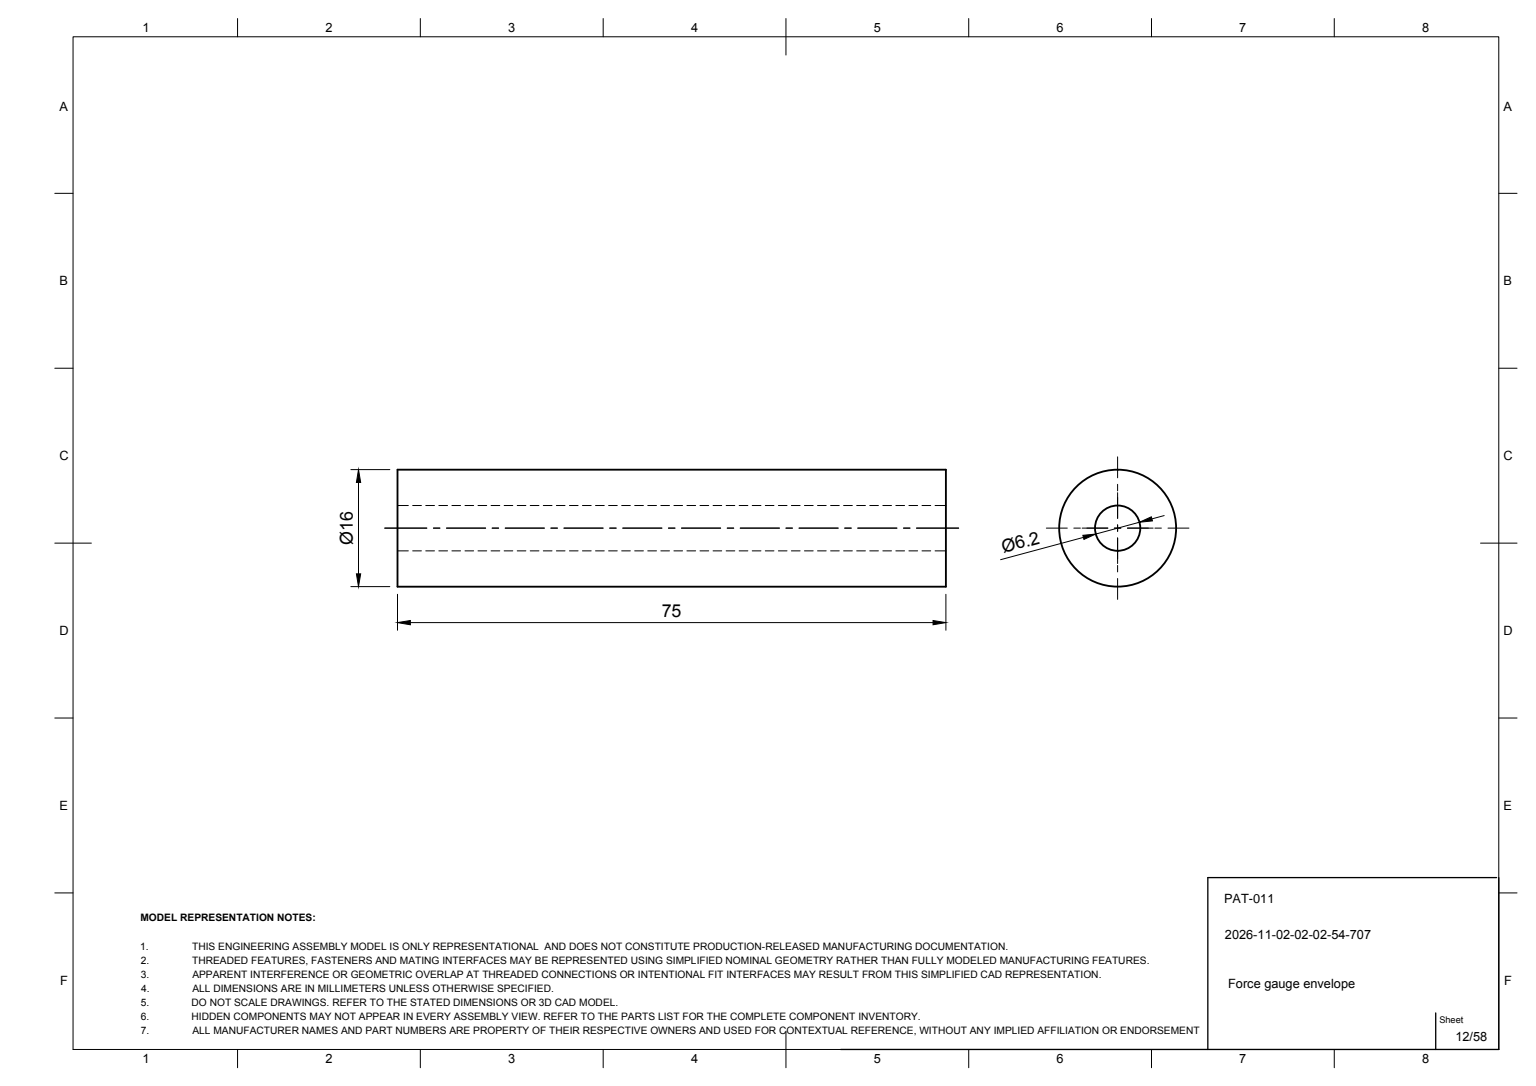
ISO-10303-21;
HEADER;
/* Generated by software containing ST-Developer
 * from STEP Tools, Inc. (www.steptools.com) 
 */

FILE_DESCRIPTION(
/* description */ ('Belt tension measurement rig'),
/* implementation_level */ '2;1');

FILE_NAME(
/* name */ 'Force gauge envelope.step',
/* time_stamp */ '2026-10-28T03:24:44-07:00',
/* author */ (''),
/* organization */ (''),
/* preprocessor_version */ 'ST-DEVELOPER v20.2',
/* originating_system */ 'Autodesk Translation Framework v15.17.0.0',
/* authorisation */ '');

FILE_SCHEMA (('AUTOMOTIVE_DESIGN { 1 0 10303 214 3 1 1 }'));
ENDSEC;

DATA;
#10=MECHANICAL_DESIGN_GEOMETRIC_PRESENTATION_REPRESENTATION('',(#703),#23587);
#593=SHAPE_REPRESENTATION_RELATIONSHIP('SRR','None',#23838,#648);
#648=ADVANCED_BREP_SHAPE_REPRESENTATION('',(#773),#23536);
#703=STYLED_ITEM('',(#24225),#773);
#773=MANIFOLD_SOLID_BREP('Body1',#12208);
#889=FACE_BOUND('',#2248,.T.);
#890=FACE_BOUND('',#2250,.T.);
#1107=PLANE('',#13143);
#1108=PLANE('',#13144);
#1481=FACE_OUTER_BOUND('',#2245,.T.);
#1482=FACE_OUTER_BOUND('',#2246,.T.);
#1483=FACE_OUTER_BOUND('',#2247,.T.);
#1484=FACE_OUTER_BOUND('',#2249,.T.);
#2245=EDGE_LOOP('',(#8460,#8461,#8462,#8463));
#2246=EDGE_LOOP('',(#8464,#8465,#8466,#8467));
#2247=EDGE_LOOP('',(#8468));
#2248=EDGE_LOOP('',(#8469));
#2249=EDGE_LOOP('',(#8470));
#2250=EDGE_LOOP('',(#8471));
#3111=LINE('',#19132,#3862);
#3112=LINE('',#19138,#3863);
#3862=VECTOR('',#15186,0.31);
#3863=VECTOR('',#15193,0.8);
#4588=CIRCLE('',#13138,0.31);
#4589=CIRCLE('',#13139,0.31);
#4590=CIRCLE('',#13141,0.8);
#4591=CIRCLE('',#13142,0.8);
#5412=VERTEX_POINT('',#19129);
#5413=VERTEX_POINT('',#19131);
#5414=VERTEX_POINT('',#19135);
#5415=VERTEX_POINT('',#19137);
#6589=EDGE_CURVE('',#5412,#5412,#4588,.T.);
#6590=EDGE_CURVE('',#5412,#5413,#3111,.T.);
#6591=EDGE_CURVE('',#5413,#5413,#4589,.T.);
#6592=EDGE_CURVE('',#5414,#5414,#4590,.T.);
#6593=EDGE_CURVE('',#5414,#5415,#3112,.T.);
#6594=EDGE_CURVE('',#5415,#5415,#4591,.T.);
#8460=ORIENTED_EDGE('',*,*,#6589,.F.);
#8461=ORIENTED_EDGE('',*,*,#6590,.T.);
#8462=ORIENTED_EDGE('',*,*,#6591,.T.);
#8463=ORIENTED_EDGE('',*,*,#6590,.F.);
#8464=ORIENTED_EDGE('',*,*,#6592,.F.);
#8465=ORIENTED_EDGE('',*,*,#6593,.T.);
#8466=ORIENTED_EDGE('',*,*,#6594,.T.);
#8467=ORIENTED_EDGE('',*,*,#6593,.F.);
#8468=ORIENTED_EDGE('',*,*,#6592,.T.);
#8469=ORIENTED_EDGE('',*,*,#6589,.T.);
#8470=ORIENTED_EDGE('',*,*,#6594,.F.);
#8471=ORIENTED_EDGE('',*,*,#6591,.F.);
#11217=CYLINDRICAL_SURFACE('',#13137,0.31);
#11218=CYLINDRICAL_SURFACE('',#13140,0.8);
#11622=ADVANCED_FACE('',(#1481),#11217,.F.);
#11623=ADVANCED_FACE('',(#1482),#11218,.T.);
#11624=ADVANCED_FACE('',(#1483,#889),#1107,.T.);
#11625=ADVANCED_FACE('',(#1484,#890),#1108,.F.);
#12208=CLOSED_SHELL('',(#11622,#11623,#11624,#11625));
#13136=AXIS2_PLACEMENT_3D('',#19127,#15180,#15181);
#13137=AXIS2_PLACEMENT_3D('',#19128,#15182,#15183);
#13138=AXIS2_PLACEMENT_3D('',#19130,#15184,#15185);
#13139=AXIS2_PLACEMENT_3D('',#19133,#15187,#15188);
#13140=AXIS2_PLACEMENT_3D('',#19134,#15189,#15190);
#13141=AXIS2_PLACEMENT_3D('',#19136,#15191,#15192);
#13142=AXIS2_PLACEMENT_3D('',#19139,#15194,#15195);
#13143=AXIS2_PLACEMENT_3D('',#19140,#15196,#15197);
#13144=AXIS2_PLACEMENT_3D('',#19141,#15198,#15199);
#15180=DIRECTION('axis',(0.,0.,1.));
#15181=DIRECTION('refdir',(1.,0.,0.));
#15182=DIRECTION('center_axis',(1.,0.,0.));
#15183=DIRECTION('ref_axis',(0.,0.,-1.));
#15184=DIRECTION('center_axis',(-1.,0.,0.));
#15185=DIRECTION('ref_axis',(0.,0.,-1.));
#15186=DIRECTION('',(-1.,0.,0.));
#15187=DIRECTION('center_axis',(-1.,0.,0.));
#15188=DIRECTION('ref_axis',(0.,0.,-1.));
#15189=DIRECTION('center_axis',(1.,0.,0.));
#15190=DIRECTION('ref_axis',(0.,0.,-1.));
#15191=DIRECTION('center_axis',(1.,0.,0.));
#15192=DIRECTION('ref_axis',(0.,0.,-1.));
#15193=DIRECTION('',(-1.,0.,0.));
#15194=DIRECTION('center_axis',(1.,0.,0.));
#15195=DIRECTION('ref_axis',(0.,0.,-1.));
#15196=DIRECTION('center_axis',(1.,0.,0.));
#15197=DIRECTION('ref_axis',(0.,0.,-1.));
#15198=DIRECTION('center_axis',(1.,0.,0.));
#15199=DIRECTION('ref_axis',(0.,0.,-1.));
#19127=CARTESIAN_POINT('',(0.,0.,0.));
#19128=CARTESIAN_POINT('Origin',(2.,7.5,4.5));
#19129=CARTESIAN_POINT('',(9.5,7.5,4.81));
#19130=CARTESIAN_POINT('Origin',(9.5,7.5,4.5));
#19131=CARTESIAN_POINT('',(2.,7.5,4.81));
#19132=CARTESIAN_POINT('',(2.,7.5,4.81));
#19133=CARTESIAN_POINT('Origin',(2.,7.5,4.5));
#19134=CARTESIAN_POINT('Origin',(2.,7.5,4.5));
#19135=CARTESIAN_POINT('',(9.5,7.5,5.3));
#19136=CARTESIAN_POINT('Origin',(9.5,7.5,4.5));
#19137=CARTESIAN_POINT('',(2.,7.5,5.3));
#19138=CARTESIAN_POINT('',(2.,7.5,5.3));
#19139=CARTESIAN_POINT('Origin',(2.,7.5,4.5));
#19140=CARTESIAN_POINT('Origin',(9.5,7.5,4.5));
#19141=CARTESIAN_POINT('Origin',(2.,7.5,4.5));
#23471=UNCERTAINTY_MEASURE_WITH_UNIT(LENGTH_MEASURE(0.001),#23588,
'DISTANCE_ACCURACY_VALUE',
'Maximum model space distance between geometric entities at asserted c
onnectivities');
#23522=UNCERTAINTY_MEASURE_WITH_UNIT(LENGTH_MEASURE(0.001),#23588,
'DISTANCE_ACCURACY_VALUE',
'Maximum model space distance between geometric entities at asserted c
onnectivities');
#23536=(
GEOMETRIC_REPRESENTATION_CONTEXT(3)
GLOBAL_UNCERTAINTY_ASSIGNED_CONTEXT((#23471))
GLOBAL_UNIT_ASSIGNED_CONTEXT((#23588,#23590,#23591))
REPRESENTATION_CONTEXT('','3D')
);
#23587=(
GEOMETRIC_REPRESENTATION_CONTEXT(3)
GLOBAL_UNCERTAINTY_ASSIGNED_CONTEXT((#23522))
GLOBAL_UNIT_ASSIGNED_CONTEXT((#23588,#23590,#23591))
REPRESENTATION_CONTEXT('','3D')
);
#23588=(
LENGTH_UNIT()
NAMED_UNIT(*)
SI_UNIT(.CENTI.,.METRE.)
);
#23590=(
NAMED_UNIT(*)
PLANE_ANGLE_UNIT()
SI_UNIT($,.RADIAN.)
);
#23591=(
NAMED_UNIT(*)
SI_UNIT($,.STERADIAN.)
SOLID_ANGLE_UNIT()
);
#23605=SHAPE_DEFINITION_REPRESENTATION(#23669,#23838);
#23669=PRODUCT_DEFINITION_SHAPE('',$,#23903);
#23838=SHAPE_REPRESENTATION('',(#13136),#23536);
#23889=PRODUCT_DEFINITION_CONTEXT('part definition',#24083,'design');
#23903=PRODUCT_DEFINITION('Force gauge envelope','Force gauge envelope',
#23967,#23889);
#23967=PRODUCT_DEFINITION_FORMATION('',$,#24098);
#24083=APPLICATION_CONTEXT(
'Core Data for Automotive Mechanical Design Process');
#24084=PRODUCT_CONTEXT('part definition',#24083,'mechanical');
#24098=PRODUCT('Force gauge envelope','Force gauge envelope',
'Force gauge envelope',(#24084));
#24219=COLOUR_RGB('Off White',0.89,0.88,0.83);
#24220=FILL_AREA_STYLE_COLOUR('',#24219);
#24221=FILL_AREA_STYLE('',(#24220));
#24222=SURFACE_STYLE_FILL_AREA(#24221);
#24223=SURFACE_SIDE_STYLE('',(#24222));
#24224=SURFACE_STYLE_USAGE(.BOTH.,#24223);
#24225=PRESENTATION_STYLE_ASSIGNMENT((#24224));
ENDSEC;
END-ISO-10303-21;
